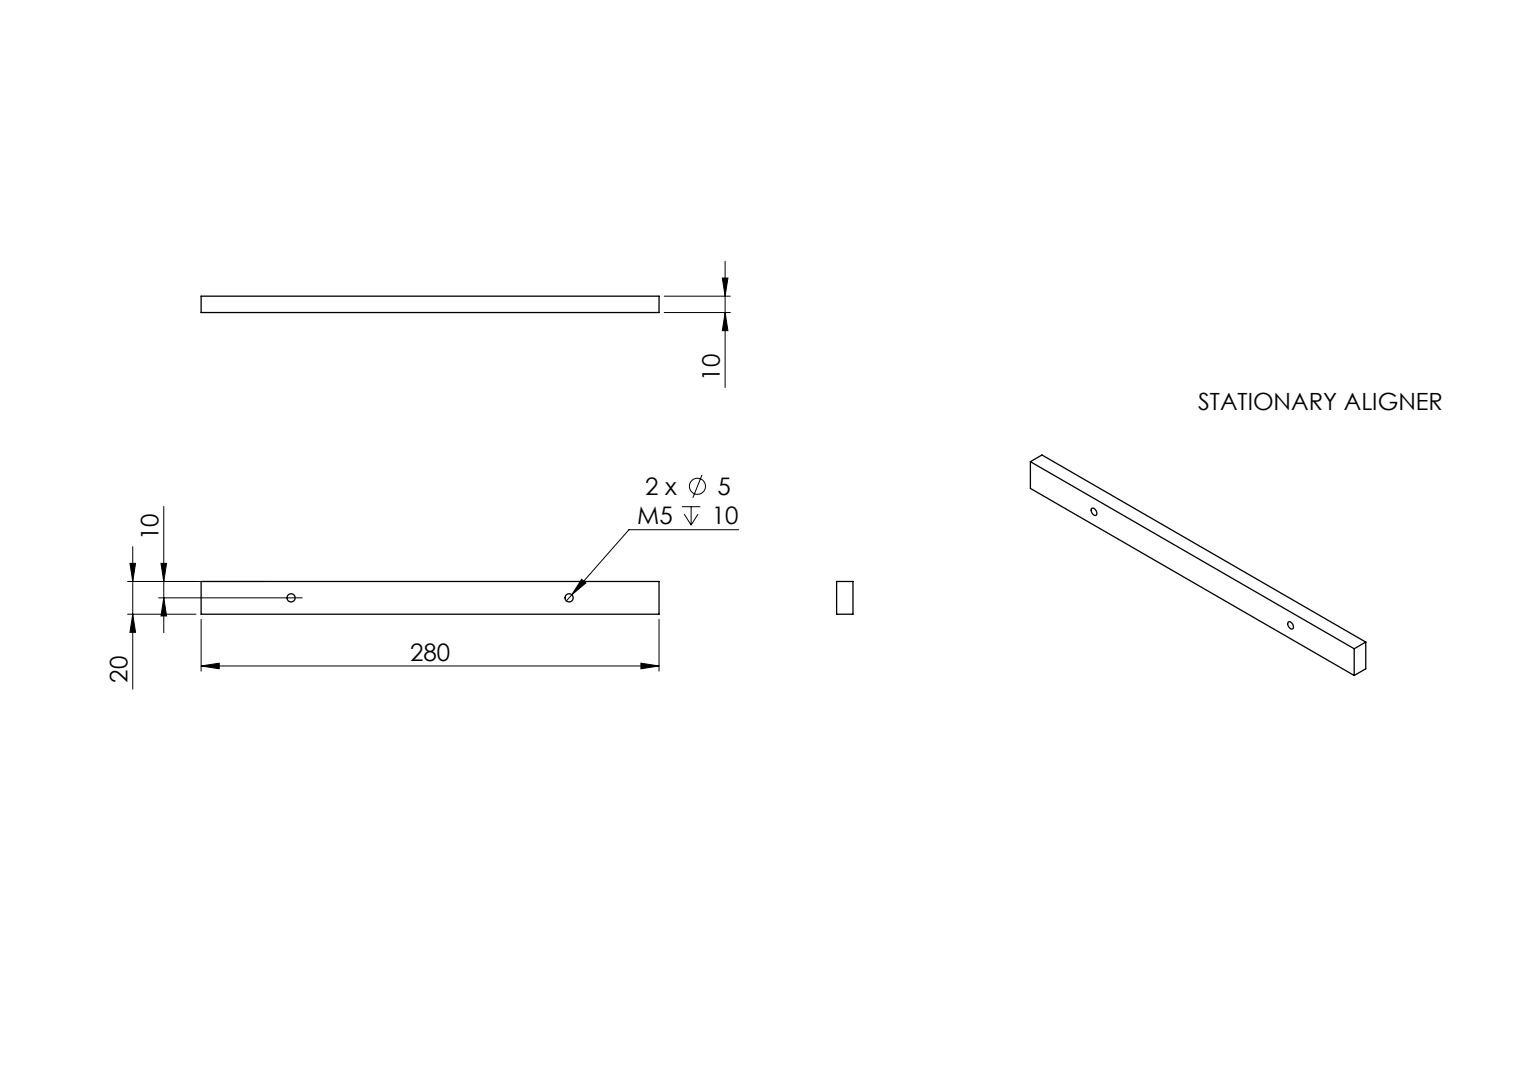
ISO-10303-21;
HEADER;
FILE_DESCRIPTION (('STEP AP214'),
    '1' );
FILE_NAME ('stationary aligner.step',
    '2026-10-24T13:33:06',
    ( '' ),
    ( '' ),
    'SwSTEP 2.0',
    'SolidWorks 2026',
    '' );
FILE_SCHEMA (( 'AUTOMOTIVE_DESIGN' ));
ENDSEC;

DATA;
#35=( GEOMETRIC_REPRESENTATION_CONTEXT ( 3 ) GLOBAL_UNCERTAINTY_ASSIGNED_CONTEXT ( ( #12045 ) ) GLOBAL_UNIT_ASSIGNED_CONTEXT ( ( #1891, #1958, #13996 ) ) REPRESENTATION_CONTEXT ( 'NONE', 'WORKASPACE' ) );
#50=VERTEX_POINT ( 'NONE', #7335 ) ;
#53=ORIENTED_EDGE ( 'NONE', *, *, #841, .T. ) ;
#69=ORIENTED_EDGE ( 'NONE', *, *, #9344, .T. ) ;
#97=LINE ( 'NONE', #13393, #5781 ) ;
#217=PLANE ( 'NONE',  #14054 ) ;
#315=CARTESIAN_POINT ( 'NONE',  ( 304.9999999999999432, 45.00000000000001421, 0.000000000000000000 ) ) ;
#345=ORIENTED_EDGE ( 'NONE', *, *, #12797, .F. ) ;
#350=ORIENTED_EDGE ( 'NONE', *, *, #717, .F. ) ;
#355=CARTESIAN_POINT ( 'NONE',  ( 79.99999999999971578, 55.00000000000000711, 0.000000000000000000 ) ) ;
#399=CARTESIAN_POINT ( 'NONE',  ( 132.4999999999999716, 45.00000000000001421, 10.00000000000000000 ) ) ;
#425=LINE ( 'NONE', #10396, #7577 ) ;
#459=CIRCLE ( 'NONE', #14158, 2.500000000000002220 ) ;
#469=CARTESIAN_POINT ( 'NONE',  ( 307.4999999999999432, 45.00000000000001421, 10.00000000000000000 ) ) ;
#536=ORIENTED_EDGE ( 'NONE', *, *, #14163, .F. ) ;
#573=DIRECTION ( 'NONE',  ( -0.000000000000000000, -0.000000000000000000, -1.000000000000000000 ) ) ;
#584=EDGE_CURVE ( 'NONE', #2928, #10867, #1475, .T. ) ;
#605=APPLICATION_CONTEXT ( 'automotive_design' ) ;
#653=FACE_OUTER_BOUND ( 'NONE', #14300, .T. ) ;
#672=STYLED_ITEM('',(#14403),#3882);
#679=CARTESIAN_POINT ( 'NONE',  ( 359.9999999999997726, 35.00000000000002842, 0.000000000000000000 ) ) ;
#690=AXIS2_PLACEMENT_3D ( 'NONE', #8292, #2793, #13735 ) ;
#717=EDGE_CURVE ( 'NONE', #7761, #2624, #1126, .T. ) ;
#767=ORIENTED_EDGE ( 'NONE', *, *, #841, .F. ) ;
#780=SURFACE_SIDE_STYLE ('',( #7408 ) ) ;
#841=EDGE_CURVE ( 'NONE', #7650, #1100, #97, .T. ) ;
#874=DIRECTION ( 'NONE',  ( -1.000000000000000000, 0.000000000000000000, -0.000000000000000000 ) ) ;
#1062=AXIS2_PLACEMENT_3D ( 'NONE', #12681, #2536, #5795 ) ;
#1100=VERTEX_POINT ( 'NONE', #679 ) ;
#1126=LINE ( 'NONE', #3408, #12403 ) ;
#1244=VERTEX_POINT ( 'NONE', #10316 ) ;
#1284=DIRECTION ( 'NONE',  ( -0.000000000000000000, -0.000000000000000000, -1.000000000000000000 ) ) ;
#1383=EDGE_LOOP ( 'NONE', ( #345, #4105, #13861, #8280 ) ) ;
#1431=EDGE_CURVE ( 'NONE', #1100, #50, #10979, .T. ) ;
#1458=ORIENTED_EDGE ( 'NONE', *, *, #9714, .T. ) ;
#1475=CIRCLE ( 'NONE', #5894, 2.500000000000002220 ) ;
#1708=VERTEX_POINT ( 'NONE', #399 ) ;
#1735=CARTESIAN_POINT ( 'NONE',  ( 79.99999999999971578, 35.00000000000000000, 0.000000000000000000 ) ) ;
#1818=DIRECTION ( 'NONE',  ( 1.000000000000000000, 9.912705577010325549E-17, 0.000000000000000000 ) ) ;
#1821=EDGE_LOOP ( 'NONE', ( #3567, #69 ) ) ;
#1831=DIRECTION ( 'NONE',  ( -1.000000000000000000, -2.478176394252579230E-17, -0.000000000000000000 ) ) ;
#1871=DIRECTION ( 'NONE',  ( -0.000000000000000000, -0.000000000000000000, -1.000000000000000000 ) ) ;
#1891=( LENGTH_UNIT ( ) NAMED_UNIT ( * ) SI_UNIT ( .MILLI., .METRE. ) );
#1958=( NAMED_UNIT ( * ) PLANE_ANGLE_UNIT ( ) SI_UNIT ( $, .RADIAN. ) );
#1981=FACE_BOUND ( 'NONE', #1821, .T. ) ;
#2007=PLANE ( 'NONE',  #6419 ) ;
#2008=VECTOR ( 'NONE', #8358, 1000.000000000000000 ) ;
#2030=CIRCLE ( 'NONE', #5739, 2.500000000000002220 ) ;
#2083=FACE_OUTER_BOUND ( 'NONE', #13848, .T. ) ;
#2199=FACE_BOUND ( 'NONE', #9232, .T. ) ;
#2354=ORIENTED_EDGE ( 'NONE', *, *, #6579, .T. ) ;
#2420=ORIENTED_EDGE ( 'NONE', *, *, #8634, .T. ) ;
#2436=CARTESIAN_POINT ( 'NONE',  ( 79.99999999999971578, 35.00000000000000000, 10.00000000000000000 ) ) ;
#2457=CARTESIAN_POINT ( 'NONE',  ( 134.9999999999999716, 45.00000000000001421, 0.000000000000000000 ) ) ;
#2475=DIRECTION ( 'NONE',  ( 1.000000000000000000, 2.478176394252579538E-17, 0.000000000000000000 ) ) ;
#2516=DIRECTION ( 'NONE',  ( -1.000000000000000000, 0.000000000000000000, 0.000000000000000000 ) ) ;
#2536=DIRECTION ( 'NONE',  ( -9.912705577010325549E-17, 1.000000000000000000, 0.000000000000000000 ) ) ;
#2575=CIRCLE ( 'NONE', #690, 2.500000000000002220 ) ;
#2624=VERTEX_POINT ( 'NONE', #8124 ) ;
#2641=CARTESIAN_POINT ( 'NONE',  ( 79.99999999999971578, 55.00000000000000711, 10.00000000000000000 ) ) ;
#2709=VECTOR ( 'NONE', #2970, 1000.000000000000000 ) ;
#2793=DIRECTION ( 'NONE',  ( -0.000000000000000000, -0.000000000000000000, -1.000000000000000000 ) ) ;
#2928=VERTEX_POINT ( 'NONE', #8641 ) ;
#2970=DIRECTION ( 'NONE',  ( -0.000000000000000000, -0.000000000000000000, -1.000000000000000000 ) ) ;
#3038=CARTESIAN_POINT ( 'NONE',  ( 132.4999999999999716, 45.00000000000001421, 0.000000000000000000 ) ) ;
#3183=VECTOR ( 'NONE', #7058, 1000.000000000000000 ) ;
#3188=LINE ( 'NONE', #6368, #2709 ) ;
#3206=UNCERTAINTY_MEASURE_WITH_UNIT (LENGTH_MEASURE( 1.000000000000000082E-05 ), #12844, 'distance_accuracy_value', 'NONE');
#3236=CARTESIAN_POINT ( 'NONE',  ( 0.000000000000000000, 0.000000000000000000, 10.00000000000000000 ) ) ;
#3245=ORIENTED_EDGE ( 'NONE', *, *, #8825, .T. ) ;
#3408=CARTESIAN_POINT ( 'NONE',  ( 79.99999999999971578, 35.00000000000000000, 0.000000000000000000 ) ) ;
#3416=CARTESIAN_POINT ( 'NONE',  ( 307.4999999999999432, 45.00000000000001421, 0.000000000000000000 ) ) ;
#3548=EDGE_CURVE ( 'NONE', #1708, #10304, #2575, .T. ) ;
#3567=ORIENTED_EDGE ( 'NONE', *, *, #3548, .T. ) ;
#3586=ORIENTED_EDGE ( 'NONE', *, *, #8634, .F. ) ;
#3653=CIRCLE ( 'NONE', #4820, 2.500000000000002220 ) ;
#3656=ORIENTED_EDGE ( 'NONE', *, *, #13239, .T. ) ;
#3695=FACE_OUTER_BOUND ( 'NONE', #13057, .T. ) ;
#3755=ORIENTED_EDGE ( 'NONE', *, *, #9883, .T. ) ;
#3766=DIRECTION ( 'NONE',  ( -1.000000000000000000, -2.478176394252579230E-17, -0.000000000000000000 ) ) ;
#3794=EDGE_LOOP ( 'NONE', ( #12275, #2354, #2420, #13391 ) ) ;
#3858=ORIENTED_EDGE ( 'NONE', *, *, #8825, .F. ) ;
#3882=MANIFOLD_SOLID_BREP ( 'AdvancedHole1', #12608 ) ;
#3925=EDGE_CURVE ( 'NONE', #13016, #7650, #4072, .T. ) ;
#3994=DIRECTION ( 'NONE',  ( -0.000000000000000000, -0.000000000000000000, -1.000000000000000000 ) ) ;
#4041=ADVANCED_BREP_SHAPE_REPRESENTATION ( '', ( #3882, #14039 ), #35 ) ;
#4047=DIRECTION ( 'NONE',  ( -0.000000000000000000, -0.000000000000000000, -1.000000000000000000 ) ) ;
#4072=LINE ( 'NONE', #7481, #5345 ) ;
#4105=ORIENTED_EDGE ( 'NONE', *, *, #3548, .F. ) ;
#4116=ORIENTED_EDGE ( 'NONE', *, *, #12433, .F. ) ;
#4122=VECTOR ( 'NONE', #3994, 1000.000000000000000 ) ;
#4125=CARTESIAN_POINT ( 'NONE',  ( 359.9999999999997726, 35.00000000000002842, 10.00000000000000000 ) ) ;
#4127=PRODUCT_DEFINITION_CONTEXT ( 'detailed design', #9055, 'design' ) ;
#4156=VERTEX_POINT ( 'NONE', #469 ) ;
#4161=UNCERTAINTY_MEASURE_WITH_UNIT (LENGTH_MEASURE( 1.000000000000000082E-05 ), #7540, 'distance_accuracy_value', 'NONE');
#4199=ADVANCED_FACE ( 'NONE', ( #3695 ), #7031, .F. ) ;
#4220=SURFACE_STYLE_USAGE ( .BOTH. , #780 ) ;
#4222=( NAMED_UNIT ( * ) PLANE_ANGLE_UNIT ( ) SI_UNIT ( $, .RADIAN. ) );
#4229=SHAPE_REPRESENTATION ( 'stationary aligner', ( #14039 ), #35 ) ;
#4233=VECTOR ( 'NONE', #3766, 1000.000000000000000 ) ;
#4236=LINE ( 'NONE', #7196, #2008 ) ;
#4262=ORIENTED_EDGE ( 'NONE', *, *, #13239, .F. ) ;
#4311=FACE_OUTER_BOUND ( 'NONE', #3794, .T. ) ;
#4320=ORIENTED_EDGE ( 'NONE', *, *, #9344, .F. ) ;
#4332=CIRCLE ( 'NONE', #6180, 2.500000000000002220 ) ;
#4335=VECTOR ( 'NONE', #6103, 1000.000000000000000 ) ;
#4340=LINE ( 'NONE', #8761, #12199 ) ;
#4368=EDGE_CURVE ( 'NONE', #9829, #50, #7384, .T. ) ;
#4371=ORIENTED_EDGE ( 'NONE', *, *, #4368, .F. ) ;
#4477=PRODUCT_DEFINITION_FORMATION_WITH_SPECIFIED_SOURCE ( 'ANY', '', #10055, .NOT_KNOWN. ) ;
#4559=DIRECTION ( 'NONE',  ( -0.000000000000000000, -0.000000000000000000, -1.000000000000000000 ) ) ;
#4581=AXIS2_PLACEMENT_3D ( 'NONE', #9756, #10915, #13230 ) ;
#4656=EDGE_LOOP ( 'NONE', ( #8216, #3245, #3755, #8712 ) ) ;
#4820=AXIS2_PLACEMENT_3D ( 'NONE', #9802, #7607, #13199 ) ;
#4908=STYLED_ITEM ( 'NONE', ( #9662 ), #4041 ) ;
#4942=DIRECTION ( 'NONE',  ( -0.000000000000000000, -0.000000000000000000, -1.000000000000000000 ) ) ;
#4944=AXIS2_PLACEMENT_3D ( 'NONE', #12762, #4942, #13844 ) ;
#5001=FACE_OUTER_BOUND ( 'NONE', #6397, .T. ) ;
#5077=DIRECTION ( 'NONE',  ( 1.000000000000000000, 0.000000000000000000, 0.000000000000000000 ) ) ;
#5089=CARTESIAN_POINT ( 'NONE',  ( 137.4999999999999716, 45.00000000000001421, 0.000000000000000000 ) ) ;
#5116=DIRECTION ( 'NONE',  ( -1.000000000000000000, 0.000000000000000000, 0.000000000000000000 ) ) ;
#5156=VECTOR ( 'NONE', #7277, 1000.000000000000000 ) ;
#5302=DIRECTION ( 'NONE',  ( -0.000000000000000000, -0.000000000000000000, -1.000000000000000000 ) ) ;
#5345=VECTOR ( 'NONE', #1818, 1000.000000000000000 ) ;
#5379=FILL_AREA_STYLE ('',( #14215 ) ) ;
#5407=ADVANCED_FACE ( 'NONE', ( #8731 ), #11934, .F. ) ;
#5415=CARTESIAN_POINT ( 'NONE',  ( 134.9999999999999716, 45.00000000000001421, 10.00000000000000000 ) ) ;
#5419=ADVANCED_FACE ( 'NONE', ( #1981, #2199, #4311 ), #13293, .F. ) ;
#5444=CARTESIAN_POINT ( 'NONE',  ( 302.4999999999999432, 45.00000000000001421, 0.000000000000000000 ) ) ;
#5515=LINE ( 'NONE', #5846, #9202 ) ;
#5603=CARTESIAN_POINT ( 'NONE',  ( 79.99999999999971578, 55.00000000000000711, 10.00000000000000000 ) ) ;
#5638=CARTESIAN_POINT ( 'NONE',  ( 304.9999999999999432, 45.00000000000001421, 10.00000000000000000 ) ) ;
#5739=AXIS2_PLACEMENT_3D ( 'NONE', #8525, #14172, #13167 ) ;
#5781=VECTOR ( 'NONE', #4559, 1000.000000000000000 ) ;
#5792=DIRECTION ( 'NONE',  ( -0.000000000000000000, -1.000000000000000000, -0.000000000000000000 ) ) ;
#5795=DIRECTION ( 'NONE',  ( -1.000000000000000000, -9.912705577010325549E-17, 0.000000000000000000 ) ) ;
#5805=VECTOR ( 'NONE', #4047, 1000.000000000000000 ) ;
#5830=FACE_BOUND ( 'NONE', #7021, .T. ) ;
#5846=CARTESIAN_POINT ( 'NONE',  ( 79.99999999999971578, 35.00000000000000000, 10.00000000000000000 ) ) ;
#5859=ADVANCED_FACE ( 'NONE', ( #11983 ), #12123, .F. ) ;
#5867=CARTESIAN_POINT ( 'NONE',  ( 360.0000000000000000, 55.00000000000001421, 10.00000000000000000 ) ) ;
#5894=AXIS2_PLACEMENT_3D ( 'NONE', #7526, #5302, #10739 ) ;
#5897=EDGE_LOOP ( 'NONE', ( #13879, #7656, #3586, #8202 ) ) ;
#6103=DIRECTION ( 'NONE',  ( 1.000000000000000000, 9.912705577010325549E-17, 0.000000000000000000 ) ) ;
#6115=CYLINDRICAL_SURFACE ( 'NONE', #11283, 2.500000000000002220 ) ;
#6180=AXIS2_PLACEMENT_3D ( 'NONE', #2457, #11385, #6882 ) ;
#6323=ADVANCED_FACE ( 'NONE', ( #5001 ), #8176, .F. ) ;
#6335=EDGE_CURVE ( 'NONE', #10867, #2928, #4332, .T. ) ;
#6368=CARTESIAN_POINT ( 'NONE',  ( 79.99999999999971578, 35.00000000000000000, 10.00000000000000000 ) ) ;
#6397=EDGE_LOOP ( 'NONE', ( #12782, #767, #10521, #13988 ) ) ;
#6419=AXIS2_PLACEMENT_3D ( 'NONE', #6515, #8543, #6444 ) ;
#6444=DIRECTION ( 'NONE',  ( -1.110223024625157487E-14, -1.000000000000000000, 0.000000000000000000 ) ) ;
#6467=DIRECTION ( 'NONE',  ( -1.000000000000000000, 0.000000000000000000, 0.000000000000000000 ) ) ;
#6487=DIRECTION ( 'NONE',  ( 0.000000000000000000, 0.000000000000000000, -1.000000000000000000 ) ) ;
#6509=ADVANCED_FACE ( 'NONE', ( #13300, #5830, #6781 ), #217, .T. ) ;
#6515=CARTESIAN_POINT ( 'NONE',  ( 359.9999999999997726, 35.00000000000002842, 10.00000000000000000 ) ) ;
#6566=CARTESIAN_POINT ( 'NONE',  ( 79.99999999999971578, 55.00000000000000711, 10.00000000000000000 ) ) ;
#6579=EDGE_CURVE ( 'NONE', #9829, #10653, #425, .T. ) ;
#6698=EDGE_CURVE ( 'NONE', #10653, #7761, #12576, .T. ) ;
#6708=DIRECTION ( 'NONE',  ( -1.000000000000000000, 0.000000000000000000, -0.000000000000000000 ) ) ;
#6781=FACE_OUTER_BOUND ( 'NONE', #10534, .T. ) ;
#6790=MECHANICAL_DESIGN_GEOMETRIC_PRESENTATION_REPRESENTATION('',(#4908),#7931);
#6828=LINE ( 'NONE', #1735, #4335 ) ;
#6833=PRODUCT_DEFINITION ( 'UNKNOWN', '', #4477, #4127 ) ;
#6882=DIRECTION ( 'NONE',  ( -1.000000000000000000, 0.000000000000000000, 0.000000000000000000 ) ) ;
#6892=AXIS2_PLACEMENT_3D ( 'NONE', #13278, #9811, #6467 ) ;
#6944=ADVANCED_FACE ( 'NONE', ( #10034 ), #9144, .F. ) ;
#6952=DIRECTION ( 'NONE',  ( -0.000000000000000000, -0.000000000000000000, -1.000000000000000000 ) ) ;
#7021=EDGE_LOOP ( 'NONE', ( #4262, #12371 ) ) ;
#7031=CYLINDRICAL_SURFACE ( 'NONE', #9005, 2.500000000000002220 ) ;
#7058=DIRECTION ( 'NONE',  ( -0.000000000000000000, -0.000000000000000000, -1.000000000000000000 ) ) ;
#7195=ORIENTED_EDGE ( 'NONE', *, *, #584, .F. ) ;
#7196=CARTESIAN_POINT ( 'NONE',  ( 359.9999999999997726, 35.00000000000002842, 10.00000000000000000 ) ) ;
#7220=CIRCLE ( 'NONE', #9077, 2.500000000000002220 ) ;
#7277=DIRECTION ( 'NONE',  ( -0.000000000000000000, -0.000000000000000000, -1.000000000000000000 ) ) ;
#7335=CARTESIAN_POINT ( 'NONE',  ( 360.0000000000000000, 55.00000000000001421, 0.000000000000000000 ) ) ;
#7384=LINE ( 'NONE', #9495, #13179 ) ;
#7408=SURFACE_STYLE_FILL_AREA ( #5379 ) ;
#7419=( GEOMETRIC_REPRESENTATION_CONTEXT ( 3 ) GLOBAL_UNCERTAINTY_ASSIGNED_CONTEXT ( ( #4161 ) ) GLOBAL_UNIT_ASSIGNED_CONTEXT ( ( #7540, #4222, #14075 ) ) REPRESENTATION_CONTEXT ( 'NONE', 'WORKASPACE' ) );
#7455=DIRECTION ( 'NONE',  ( -0.000000000000000000, -0.000000000000000000, -1.000000000000000000 ) ) ;
#7481=CARTESIAN_POINT ( 'NONE',  ( 79.99999999999971578, 35.00000000000000000, 10.00000000000000000 ) ) ;
#7526=CARTESIAN_POINT ( 'NONE',  ( 134.9999999999999716, 45.00000000000001421, 0.000000000000000000 ) ) ;
#7540=( LENGTH_UNIT ( ) NAMED_UNIT ( * ) SI_UNIT ( .MILLI., .METRE. ) );
#7577=VECTOR ( 'NONE', #1831, 1000.000000000000000 ) ;
#7607=DIRECTION ( 'NONE',  ( -0.000000000000000000, -0.000000000000000000, -1.000000000000000000 ) ) ;
#7613=( NAMED_UNIT ( * ) SI_UNIT ( $, .STERADIAN. ) SOLID_ANGLE_UNIT ( ) );
#7650=VERTEX_POINT ( 'NONE', #4125 ) ;
#7656=ORIENTED_EDGE ( 'NONE', *, *, #7667, .F. ) ;
#7667=EDGE_CURVE ( 'NONE', #13016, #2624, #3188, .T. ) ;
#7716=ADVANCED_FACE ( 'NONE', ( #2083 ), #2007, .F. ) ;
#7761=VERTEX_POINT ( 'NONE', #355 ) ;
#7809=DIRECTION ( 'NONE',  ( -0.000000000000000000, -1.000000000000000000, -0.000000000000000000 ) ) ;
#7931=( GEOMETRIC_REPRESENTATION_CONTEXT ( 3 ) GLOBAL_UNCERTAINTY_ASSIGNED_CONTEXT ( ( #3206 ) ) GLOBAL_UNIT_ASSIGNED_CONTEXT ( ( #12844, #8708, #7613 ) ) REPRESENTATION_CONTEXT ( 'NONE', 'WORKASPACE' ) );
#7984=VERTEX_POINT ( 'NONE', #11781 ) ;
#8124=CARTESIAN_POINT ( 'NONE',  ( 79.99999999999971578, 35.00000000000000000, 0.000000000000000000 ) ) ;
#8176=PLANE ( 'NONE',  #1062 ) ;
#8202=ORIENTED_EDGE ( 'NONE', *, *, #6698, .T. ) ;
#8216=ORIENTED_EDGE ( 'NONE', *, *, #13054, .F. ) ;
#8226=AXIS2_PLACEMENT_3D ( 'NONE', #5603, #13555, #2475 ) ;
#8280=ORIENTED_EDGE ( 'NONE', *, *, #584, .T. ) ;
#8292=CARTESIAN_POINT ( 'NONE',  ( 134.9999999999999716, 45.00000000000001421, 10.00000000000000000 ) ) ;
#8333=EDGE_CURVE ( 'NONE', #2624, #1100, #6828, .T. ) ;
#8358=DIRECTION ( 'NONE',  ( 1.110223024625157487E-14, 1.000000000000000000, 0.000000000000000000 ) ) ;
#8525=CARTESIAN_POINT ( 'NONE',  ( 304.9999999999999432, 45.00000000000001421, 0.000000000000000000 ) ) ;
#8542=ORIENTED_EDGE ( 'NONE', *, *, #1431, .T. ) ;
#8543=DIRECTION ( 'NONE',  ( -1.000000000000000000, 1.110223024625157487E-14, 0.000000000000000000 ) ) ;
#8556=LINE ( 'NONE', #10601, #4122 ) ;
#8568=ORIENTED_EDGE ( 'NONE', *, *, #1431, .F. ) ;
#8634=EDGE_CURVE ( 'NONE', #10653, #13016, #5515, .T. ) ;
#8641=CARTESIAN_POINT ( 'NONE',  ( 132.4999999999999716, 45.00000000000001421, 0.000000000000000000 ) ) ;
#8708=( NAMED_UNIT ( * ) PLANE_ANGLE_UNIT ( ) SI_UNIT ( $, .RADIAN. ) );
#8712=ORIENTED_EDGE ( 'NONE', *, *, #9714, .F. ) ;
#8731=FACE_OUTER_BOUND ( 'NONE', #5897, .T. ) ;
#8761=CARTESIAN_POINT ( 'NONE',  ( 307.4999999999999432, 45.00000000000001421, 0.000000000000000000 ) ) ;
#8792=DIRECTION ( 'NONE',  ( 1.110223024625157487E-14, 1.000000000000000000, 0.000000000000000000 ) ) ;
#8820=DIRECTION ( 'NONE',  ( -1.000000000000000000, 0.000000000000000000, 0.000000000000000000 ) ) ;
#8825=EDGE_CURVE ( 'NONE', #4156, #14268, #4340, .T. ) ;
#8966=DIRECTION ( 'NONE',  ( -0.000000000000000000, -0.000000000000000000, -1.000000000000000000 ) ) ;
#8978=ORIENTED_EDGE ( 'NONE', *, *, #6335, .F. ) ;
#9005=AXIS2_PLACEMENT_3D ( 'NONE', #11244, #1284, #10153 ) ;
#9024=DIRECTION ( 'NONE',  ( -0.000000000000000000, -0.000000000000000000, -1.000000000000000000 ) ) ;
#9055=APPLICATION_CONTEXT ( 'automotive_design' ) ;
#9077=AXIS2_PLACEMENT_3D ( 'NONE', #315, #6952, #12470 ) ;
#9144=PLANE ( 'NONE',  #8226 ) ;
#9202=VECTOR ( 'NONE', #5792, 1000.000000000000000 ) ;
#9232=EDGE_LOOP ( 'NONE', ( #11843, #13985 ) ) ;
#9326=VECTOR ( 'NONE', #8792, 1000.000000000000000 ) ;
#9344=EDGE_CURVE ( 'NONE', #10304, #1708, #459, .T. ) ;
#9362=FACE_OUTER_BOUND ( 'NONE', #1383, .T. ) ;
#9418=DIRECTION ( 'NONE',  ( 0.000000000000000000, 0.000000000000000000, 1.000000000000000000 ) ) ;
#9472=CARTESIAN_POINT ( 'NONE',  ( 137.4999999999999716, 45.00000000000001421, 10.00000000000000000 ) ) ;
#9495=CARTESIAN_POINT ( 'NONE',  ( 360.0000000000000000, 55.00000000000001421, 10.00000000000000000 ) ) ;
#9662=PRESENTATION_STYLE_ASSIGNMENT (( #4220 ) ) ;
#9714=EDGE_CURVE ( 'NONE', #7984, #1244, #9809, .T. ) ;
#9756=CARTESIAN_POINT ( 'NONE',  ( 79.99999999999971578, 35.00000000000000000, 10.00000000000000000 ) ) ;
#9802=CARTESIAN_POINT ( 'NONE',  ( 304.9999999999999432, 45.00000000000001421, 10.00000000000000000 ) ) ;
#9809=LINE ( 'NONE', #5444, #5156 ) ;
#9811=DIRECTION ( 'NONE',  ( -0.000000000000000000, -0.000000000000000000, -1.000000000000000000 ) ) ;
#9829=VERTEX_POINT ( 'NONE', #5867 ) ;
#9883=EDGE_CURVE ( 'NONE', #14268, #1244, #7220, .T. ) ;
#9973=EDGE_CURVE ( 'NONE', #50, #7761, #12680, .T. ) ;
#9997=COLOUR_RGB ( '',0.8941176470588234615, 0.8941176470588234615, 0.8941176470588234615 ) ;
#10034=FACE_OUTER_BOUND ( 'NONE', #14061, .T. ) ;
#10055=PRODUCT ( 'stationary aligner', 'stationary aligner', '', ( #10612 ) ) ;
#10153=DIRECTION ( 'NONE',  ( -1.000000000000000000, 0.000000000000000000, 0.000000000000000000 ) ) ;
#10304=VERTEX_POINT ( 'NONE', #9472 ) ;
#10308=SHAPE_DEFINITION_REPRESENTATION ( #11097, #4229 ) ;
#10316=CARTESIAN_POINT ( 'NONE',  ( 302.4999999999999432, 45.00000000000001421, 0.000000000000000000 ) ) ;
#10396=CARTESIAN_POINT ( 'NONE',  ( 79.99999999999971578, 55.00000000000000711, 10.00000000000000000 ) ) ;
#10436=CARTESIAN_POINT ( 'NONE',  ( 79.99999999999971578, 55.00000000000000711, 0.000000000000000000 ) ) ;
#10445=CYLINDRICAL_SURFACE ( 'NONE', #4944, 2.500000000000002220 ) ;
#10464=ORIENTED_EDGE ( 'NONE', *, *, #6698, .F. ) ;
#10508=CARTESIAN_POINT ( 'NONE',  ( 0.000000000000000000, 0.000000000000000000, 0.000000000000000000 ) ) ;
#10521=ORIENTED_EDGE ( 'NONE', *, *, #3925, .F. ) ;
#10534=EDGE_LOOP ( 'NONE', ( #8568, #13933, #350, #13628 ) ) ;
#10542=CARTESIAN_POINT ( 'NONE',  ( 134.9999999999999716, 45.00000000000001421, 0.000000000000000000 ) ) ;
#10601=CARTESIAN_POINT ( 'NONE',  ( 137.4999999999999716, 45.00000000000001421, 0.000000000000000000 ) ) ;
#10612=PRODUCT_CONTEXT ( 'NONE', #605, 'mechanical' ) ;
#10653=VERTEX_POINT ( 'NONE', #6566 ) ;
#10678=ORIENTED_EDGE ( 'NONE', *, *, #9973, .T. ) ;
#10728=LINE ( 'NONE', #3038, #5805 ) ;
#10739=DIRECTION ( 'NONE',  ( -1.000000000000000000, 0.000000000000000000, 0.000000000000000000 ) ) ;
#10832=ORIENTED_EDGE ( 'NONE', *, *, #12797, .T. ) ;
#10846=ADVANCED_FACE ( 'NONE', ( #9362 ), #10445, .F. ) ;
#10867=VERTEX_POINT ( 'NONE', #5089 ) ;
#10915=DIRECTION ( 'NONE',  ( 1.000000000000000000, 0.000000000000000000, 0.000000000000000000 ) ) ;
#10979=LINE ( 'NONE', #13139, #9326 ) ;
#11097=PRODUCT_DEFINITION_SHAPE ( 'NONE', 'NONE',  #6833 ) ;
#11210=DIRECTION ( 'NONE',  ( 0.000000000000000000, 0.000000000000000000, -1.000000000000000000 ) ) ;
#11244=CARTESIAN_POINT ( 'NONE',  ( 304.9999999999999432, 45.00000000000001421, 0.000000000000000000 ) ) ;
#11283=AXIS2_PLACEMENT_3D ( 'NONE', #10542, #573, #5116 ) ;
#11381=MECHANICAL_DESIGN_GEOMETRIC_PRESENTATION_REPRESENTATION('',(#672),#7419);
#11385=DIRECTION ( 'NONE',  ( -0.000000000000000000, -0.000000000000000000, -1.000000000000000000 ) ) ;
#11387=EDGE_CURVE ( 'NONE', #1708, #2928, #10728, .T. ) ;
#11781=CARTESIAN_POINT ( 'NONE',  ( 302.4999999999999432, 45.00000000000001421, 10.00000000000000000 ) ) ;
#11843=ORIENTED_EDGE ( 'NONE', *, *, #14163, .T. ) ;
#11934=PLANE ( 'NONE',  #4581 ) ;
#11983=FACE_OUTER_BOUND ( 'NONE', #4656, .T. ) ;
#11988=ORIENTED_EDGE ( 'NONE', *, *, #11387, .F. ) ;
#12045=UNCERTAINTY_MEASURE_WITH_UNIT (LENGTH_MEASURE( 1.000000000000000082E-05 ), #1891, 'distance_accuracy_value', 'NONE');
#12123=CYLINDRICAL_SURFACE ( 'NONE', #6892, 2.500000000000002220 ) ;
#12199=VECTOR ( 'NONE', #7455, 1000.000000000000000 ) ;
#12275=ORIENTED_EDGE ( 'NONE', *, *, #12433, .T. ) ;
#12371=ORIENTED_EDGE ( 'NONE', *, *, #9883, .F. ) ;
#12403=VECTOR ( 'NONE', #7809, 1000.000000000000000 ) ;
#12405=ADVANCED_FACE ( 'NONE', ( #653 ), #6115, .F. ) ;
#12427=CARTESIAN_POINT ( 'NONE',  ( 0.000000000000000000, 0.000000000000000000, 0.000000000000000000 ) ) ;
#12433=EDGE_CURVE ( 'NONE', #7650, #9829, #4236, .T. ) ;
#12470=DIRECTION ( 'NONE',  ( -1.000000000000000000, 0.000000000000000000, 0.000000000000000000 ) ) ;
#12493=ORIENTED_EDGE ( 'NONE', *, *, #6579, .F. ) ;
#12576=LINE ( 'NONE', #2641, #3183 ) ;
#12608=CLOSED_SHELL ( 'NONE', ( #12405, #5859, #7716, #6944, #5407, #6323, #5419, #6509, #4199, #10846 ) ) ;
#12630=ORIENTED_EDGE ( 'NONE', *, *, #4368, .T. ) ;
#12669=AXIS2_PLACEMENT_3D ( 'NONE', #5638, #8966, #2516 ) ;
#12680=LINE ( 'NONE', #10436, #4233 ) ;
#12681=CARTESIAN_POINT ( 'NONE',  ( 79.99999999999971578, 35.00000000000000000, 10.00000000000000000 ) ) ;
#12683=CIRCLE ( 'NONE', #12669, 2.500000000000002220 ) ;
#12762=CARTESIAN_POINT ( 'NONE',  ( 134.9999999999999716, 45.00000000000001421, 0.000000000000000000 ) ) ;
#12782=ORIENTED_EDGE ( 'NONE', *, *, #8333, .T. ) ;
#12797=EDGE_CURVE ( 'NONE', #10304, #10867, #8556, .T. ) ;
#12844=( LENGTH_UNIT ( ) NAMED_UNIT ( * ) SI_UNIT ( .MILLI., .METRE. ) );
#13016=VERTEX_POINT ( 'NONE', #2436 ) ;
#13054=EDGE_CURVE ( 'NONE', #4156, #7984, #12683, .T. ) ;
#13057=EDGE_LOOP ( 'NONE', ( #3858, #536, #1458, #3656 ) ) ;
#13063=SHAPE_REPRESENTATION_RELATIONSHIP ( 'NONE' , 'NONE' ,  #4229, #4041 ) ;
#13139=CARTESIAN_POINT ( 'NONE',  ( 359.9999999999997726, 35.00000000000002842, 0.000000000000000000 ) ) ;
#13167=DIRECTION ( 'NONE',  ( -1.000000000000000000, 0.000000000000000000, 0.000000000000000000 ) ) ;
#13179=VECTOR ( 'NONE', #1871, 1000.000000000000000 ) ;
#13199=DIRECTION ( 'NONE',  ( -1.000000000000000000, 0.000000000000000000, 0.000000000000000000 ) ) ;
#13230=DIRECTION ( 'NONE',  ( 0.000000000000000000, 0.000000000000000000, -1.000000000000000000 ) ) ;
#13239=EDGE_CURVE ( 'NONE', #1244, #14268, #2030, .T. ) ;
#13262=EDGE_LOOP ( 'NONE', ( #7195, #8978 ) ) ;
#13278=CARTESIAN_POINT ( 'NONE',  ( 304.9999999999999432, 45.00000000000001421, 0.000000000000000000 ) ) ;
#13293=PLANE ( 'NONE',  #13830 ) ;
#13300=FACE_BOUND ( 'NONE', #13262, .T. ) ;
#13391=ORIENTED_EDGE ( 'NONE', *, *, #3925, .T. ) ;
#13393=CARTESIAN_POINT ( 'NONE',  ( 359.9999999999997726, 35.00000000000002842, 10.00000000000000000 ) ) ;
#13555=DIRECTION ( 'NONE',  ( 2.478176394252579538E-17, -1.000000000000000000, 0.000000000000000000 ) ) ;
#13628=ORIENTED_EDGE ( 'NONE', *, *, #9973, .F. ) ;
#13735=DIRECTION ( 'NONE',  ( -1.000000000000000000, 0.000000000000000000, 0.000000000000000000 ) ) ;
#13830=AXIS2_PLACEMENT_3D ( 'NONE', #3236, #6487, #874 ) ;
#13844=DIRECTION ( 'NONE',  ( -1.000000000000000000, 0.000000000000000000, 0.000000000000000000 ) ) ;
#13848=EDGE_LOOP ( 'NONE', ( #8542, #4371, #4116, #53 ) ) ;
#13861=ORIENTED_EDGE ( 'NONE', *, *, #11387, .T. ) ;
#13879=ORIENTED_EDGE ( 'NONE', *, *, #717, .T. ) ;
#13933=ORIENTED_EDGE ( 'NONE', *, *, #8333, .F. ) ;
#13985=ORIENTED_EDGE ( 'NONE', *, *, #13054, .T. ) ;
#13988=ORIENTED_EDGE ( 'NONE', *, *, #7667, .T. ) ;
#13996=( NAMED_UNIT ( * ) SI_UNIT ( $, .STERADIAN. ) SOLID_ANGLE_UNIT ( ) );
#14039=AXIS2_PLACEMENT_3D ( 'NONE', #10508, #9418, #5077 ) ;
#14054=AXIS2_PLACEMENT_3D ( 'NONE', #12427, #11210, #6708 ) ;
#14061=EDGE_LOOP ( 'NONE', ( #10678, #10464, #12493, #12630 ) ) ;
#14075=( NAMED_UNIT ( * ) SI_UNIT ( $, .STERADIAN. ) SOLID_ANGLE_UNIT ( ) );
#14158=AXIS2_PLACEMENT_3D ( 'NONE', #5415, #9024, #8820 ) ;
#14163=EDGE_CURVE ( 'NONE', #7984, #4156, #3653, .T. ) ;
#14172=DIRECTION ( 'NONE',  ( -0.000000000000000000, -0.000000000000000000, -1.000000000000000000 ) ) ;
#14215=FILL_AREA_STYLE_COLOUR ( '', #9997 ) ;
#14220=ORIENTED_EDGE ( 'NONE', *, *, #6335, .T. ) ;
#14268=VERTEX_POINT ( 'NONE', #3416 ) ;
#14300=EDGE_LOOP ( 'NONE', ( #4320, #10832, #14220, #11988 ) ) ;
#14397=COLOUR_RGB('Sky Blue',0.24,0.69,0.87);
#14398=FILL_AREA_STYLE_COLOUR('',#14397);
#14399=FILL_AREA_STYLE('',(#14398));
#14400=SURFACE_STYLE_FILL_AREA(#14399);
#14401=SURFACE_SIDE_STYLE('',(#14400));
#14402=SURFACE_STYLE_USAGE(.BOTH.,#14401);
#14403=PRESENTATION_STYLE_ASSIGNMENT((#14402));
ENDSEC;
END-ISO-10303-21;
